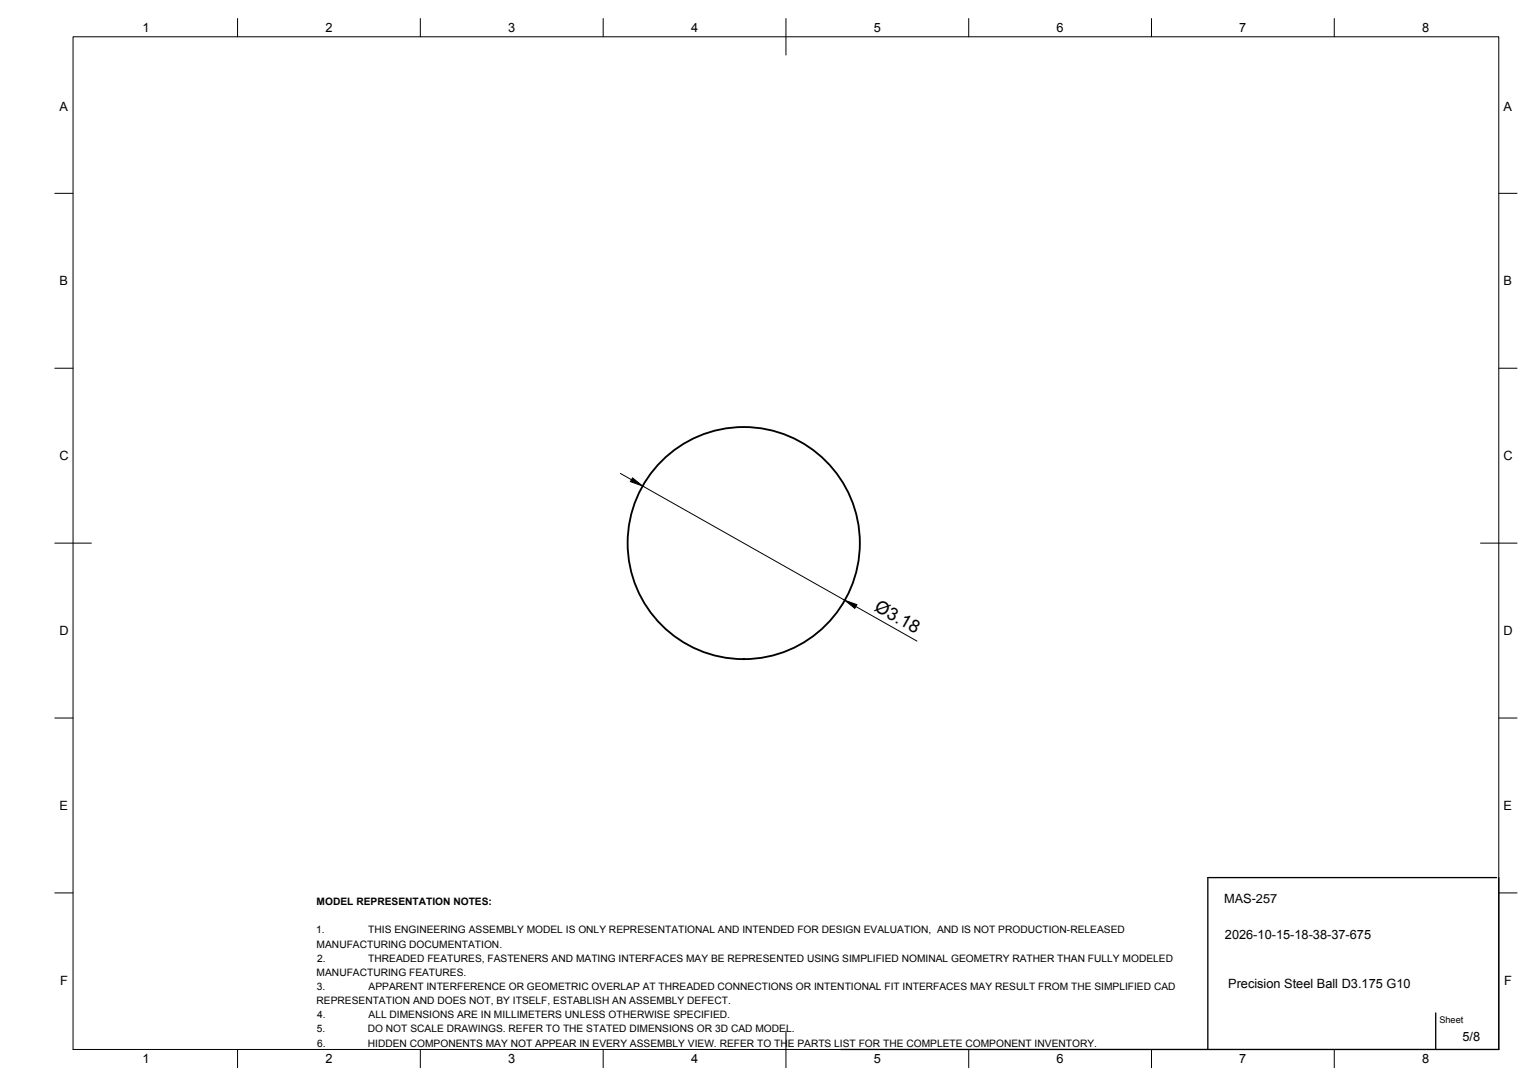
ISO-10303-21;
HEADER;
FILE_DESCRIPTION((''),'2;1');
FILE_NAME('Precision Steel Ball D3.175 G10.step','2026-10-05T22:33:56+05:00',(''),(''),'','','');
FILE_SCHEMA (('AUTOMOTIVE_DESIGN { 1 0 10303 214 3 1 1 }'));
ENDSEC;
DATA;
#10=MECHANICAL_DESIGN_GEOMETRIC_PRESENTATION_REPRESENTATION('',(#432),#16942);
#315=SPHERICAL_SURFACE('',#8594,1.5875) ;
#418=SHAPE_REPRESENTATION_RELATIONSHIP('SRR','None',#17022,#425) ;
#425=ADVANCED_BREP_SHAPE_REPRESENTATION('',(#439),#16938) ;
#432=STYLED_ITEM('',(#17066),#439) ;
#439=MANIFOLD_SOLID_BREP('Precision Steel Ball D3.175 G10',#8181) ;
#1306=FACE_OUTER_BOUND('',#1791,.T.) ;
#1791=EDGE_LOOP('',(#6625,#6626)) ;
#3273=CIRCLE('',#8595,1.5875) ;
#3819=VERTEX_POINT('',#13715) ;
#3820=VERTEX_POINT('',#13716) ;
#4810=EDGE_CURVE('',#3819,#3820,#3273,.T.) ;
#6625=ORIENTED_EDGE('',*,*,#4810,.T.) ;
#6626=ORIENTED_EDGE('',*,*,#4810,.F.) ;
#7981=ADVANCED_FACE('',(#1306),#315,.T.) ;
#8181=CLOSED_SHELL('',(#7981)) ;
#8593=AXIS2_PLACEMENT_3D('',#13713,#9923,#9924) ;
#8594=AXIS2_PLACEMENT_3D('',#13714,#9925,#9926) ;
#8595=AXIS2_PLACEMENT_3D('',#13717,#9927,#9928) ;
#9923=DIRECTION('axis',(0.,0.,1.)) ;
#9924=DIRECTION('refdir',(1.,0.,0.)) ;
#9925=DIRECTION('center_axis',(0.,0.,1.)) ;
#9926=DIRECTION('ref_axis',(1.,0.,0.)) ;
#9927=DIRECTION('center_axis',(0.,-1.,0.)) ;
#9928=DIRECTION('ref_axis',(-1.,0.,0.)) ;
#13713=CARTESIAN_POINT('',(0.,0.,0.)) ;
#13714=CARTESIAN_POINT('Origin',(35.75,31.1568542494924,31.1568542)) ;
#13715=CARTESIAN_POINT('',(35.75,31.1568542494924,32.7443542)) ;
#13716=CARTESIAN_POINT('',(35.75,31.1568542494924,29.5693542)) ;
#13717=CARTESIAN_POINT('Origin',(35.75,31.1568542494924,31.1568542)) ;
#16929=UNCERTAINTY_MEASURE_WITH_UNIT(LENGTH_MEASURE(0.01),#16943,
'DISTANCE_ACCURACY_VALUE',
'Maximum model space distance between geometric entities at asserted c
onnectivities') ;
#16933=UNCERTAINTY_MEASURE_WITH_UNIT(LENGTH_MEASURE(0.01),#16943,
'DISTANCE_ACCURACY_VALUE',
'Maximum model space distance between geometric entities at asserted c
onnectivities') ;
#16938=(
GEOMETRIC_REPRESENTATION_CONTEXT(3)
GLOBAL_UNCERTAINTY_ASSIGNED_CONTEXT((#16929))
GLOBAL_UNIT_ASSIGNED_CONTEXT((#16943,#16945,#16946))
REPRESENTATION_CONTEXT('','3D')
) ;
#16942=(
GEOMETRIC_REPRESENTATION_CONTEXT(3)
GLOBAL_UNCERTAINTY_ASSIGNED_CONTEXT((#16933))
GLOBAL_UNIT_ASSIGNED_CONTEXT((#16943,#16945,#16946))
REPRESENTATION_CONTEXT('','3D')
) ;
#16943=(
LENGTH_UNIT()
NAMED_UNIT(*)
SI_UNIT(.MILLI.,.METRE.)
) ;
#16945=(
NAMED_UNIT(*)
PLANE_ANGLE_UNIT()
SI_UNIT($,.RADIAN.)
) ;
#16946=(
NAMED_UNIT(*)
SI_UNIT($,.STERADIAN.)
SOLID_ANGLE_UNIT()
) ;
#16951=SHAPE_DEFINITION_REPRESENTATION(#16959,#17022) ;
#16959=PRODUCT_DEFINITION_SHAPE('',$,#17031) ;
#17022=SHAPE_REPRESENTATION('',(#8593),#16938) ;
#17026=PRODUCT_DEFINITION_CONTEXT('part definition',#17052,'design') ;
#17031=PRODUCT_DEFINITION('Precision Steel Ball D3.175 G10',
'Precision Steel Ball D3.175 G10',#17039,#17026) ;
#17039=PRODUCT_DEFINITION_FORMATION('',$,#17058) ;
#17052=APPLICATION_CONTEXT(
'Core Data for Automotive Mechanical Design Process') ;
#17053=PRODUCT_CONTEXT('part definition',#17052,'mechanical') ;
#17058=PRODUCT('Precision Steel Ball D3.175 G10',
'Precision Steel Ball D3.175 G10',$,(#17053)) ;
#17066=PRESENTATION_STYLE_ASSIGNMENT((#17074)) ;
#17074=SURFACE_STYLE_USAGE(.BOTH.,#17082) ;
#17082=SURFACE_SIDE_STYLE('',(#17090)) ;
#17090=SURFACE_STYLE_FILL_AREA(#17098) ;
#17098=FILL_AREA_STYLE(
'MAS-257 Metallic Sheet - Precision Steel Ball D3.175 G10',(#17106)) ;
#17106=FILL_AREA_STYLE_COLOUR(
'MAS-257 Metallic Sheet - Precision Steel Ball D3.175 G10',#17114) ;
#17114=COLOUR_RGB(
'MAS-257 Metallic Sheet - Precision Steel Ball D3.175 G10', 0.72549020, 0.75294118, 0.79215686) ;
ENDSEC;
END-ISO-10303-21;
